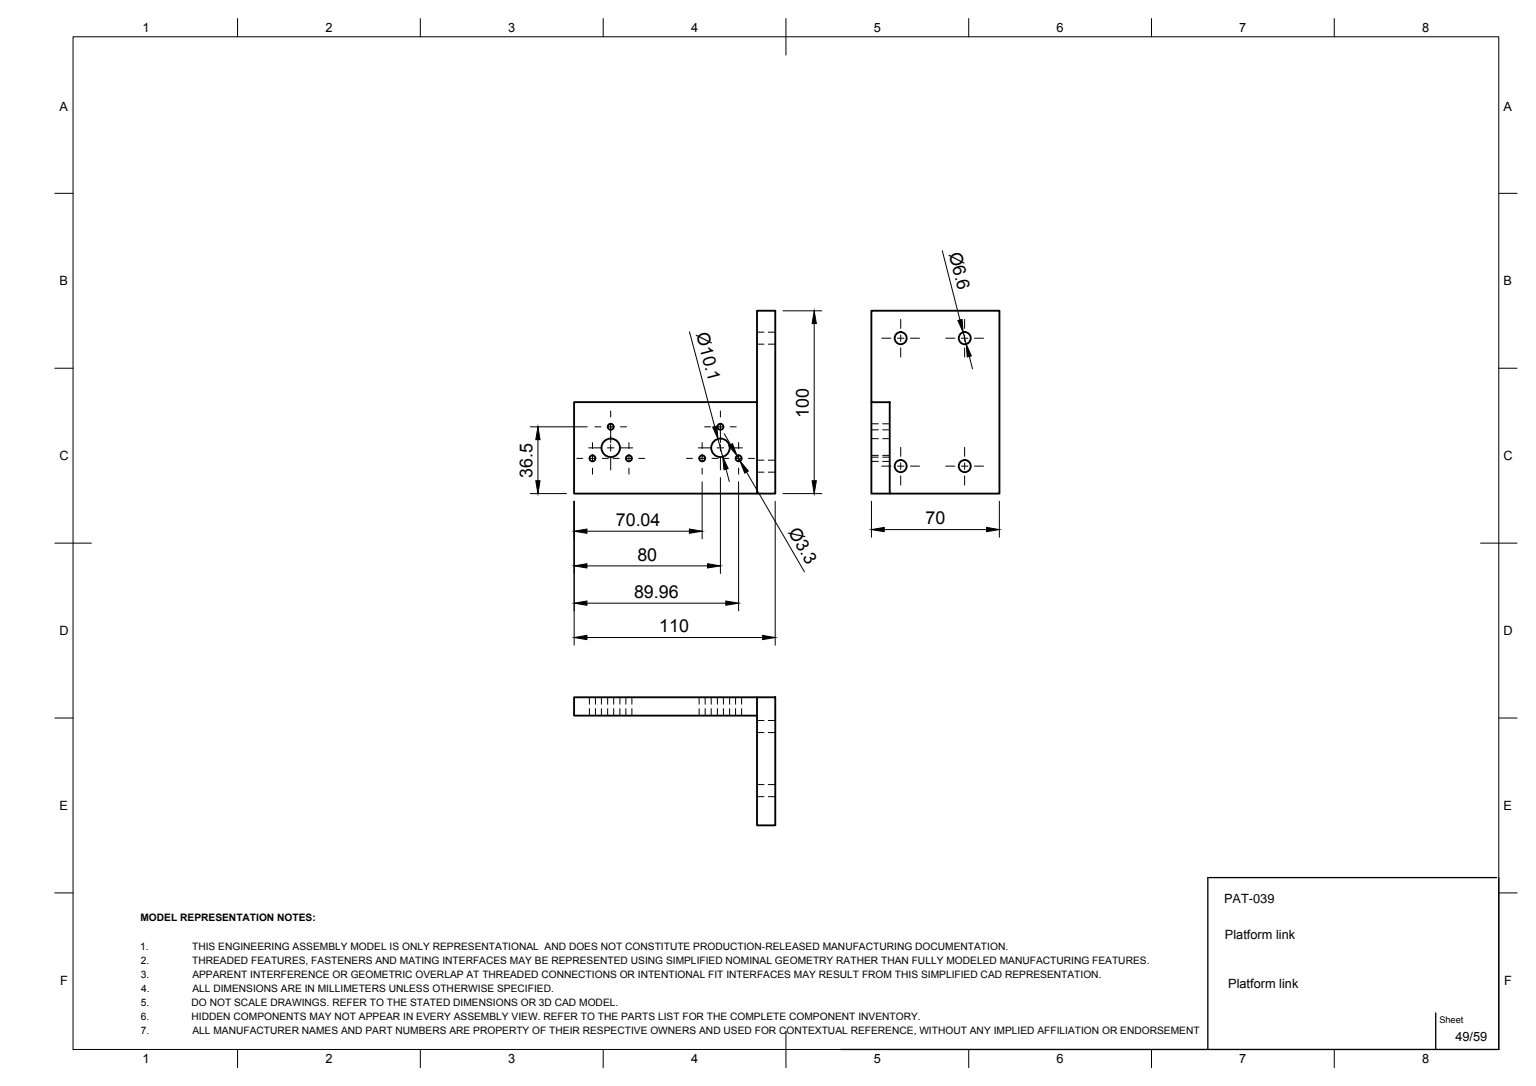
ISO-10303-21;
HEADER;
/* Generated by software containing ST-Developer
 * from STEP Tools, Inc. (www.steptools.com) 
 */

FILE_DESCRIPTION(
/* description */ ('Four-bar parallelogram arm'),
/* implementation_level */ '2;1');

FILE_NAME(
/* name */ 'Platform link.step',
/* time_stamp */ '2026-10-28T03:24:55-07:00',
/* author */ (''),
/* organization */ (''),
/* preprocessor_version */ 'ST-DEVELOPER v20.2',
/* originating_system */ 'Autodesk Translation Framework v15.17.0.0',
/* authorisation */ '');

FILE_SCHEMA (('AUTOMOTIVE_DESIGN { 1 0 10303 214 3 1 1 }'));
ENDSEC;

DATA;
#10=MECHANICAL_DESIGN_GEOMETRIC_PRESENTATION_REPRESENTATION('',(#668),#14512);
#560=SHAPE_REPRESENTATION_RELATIONSHIP('SRR','None',#14785,#610);
#610=ADVANCED_BREP_SHAPE_REPRESENTATION('',(#724),#14500);
#668=STYLED_ITEM('',(#15080),#724);
#724=MANIFOLD_SOLID_BREP('Body1',#7374);
#947=FACE_BOUND('',#2174,.T.);
#948=FACE_BOUND('',#2175,.T.);
#949=FACE_BOUND('',#2176,.T.);
#950=FACE_BOUND('',#2177,.T.);
#951=FACE_BOUND('',#2179,.T.);
#952=FACE_BOUND('',#2180,.T.);
#953=FACE_BOUND('',#2181,.T.);
#954=FACE_BOUND('',#2182,.T.);
#955=FACE_BOUND('',#2184,.T.);
#956=FACE_BOUND('',#2185,.T.);
#957=FACE_BOUND('',#2186,.T.);
#958=FACE_BOUND('',#2187,.T.);
#959=FACE_BOUND('',#2188,.T.);
#960=FACE_BOUND('',#2189,.T.);
#961=FACE_BOUND('',#2190,.T.);
#962=FACE_BOUND('',#2191,.T.);
#963=FACE_BOUND('',#2194,.T.);
#964=FACE_BOUND('',#2195,.T.);
#965=FACE_BOUND('',#2196,.T.);
#966=FACE_BOUND('',#2197,.T.);
#967=FACE_BOUND('',#2198,.T.);
#968=FACE_BOUND('',#2199,.T.);
#969=FACE_BOUND('',#2200,.T.);
#970=FACE_BOUND('',#2201,.T.);
#1155=PLANE('',#8757);
#1156=PLANE('',#8758);
#1157=PLANE('',#8759);
#1158=PLANE('',#8760);
#1159=PLANE('',#8761);
#1160=PLANE('',#8762);
#1161=PLANE('',#8763);
#1162=PLANE('',#8764);
#1163=PLANE('',#8765);
#1527=FACE_OUTER_BOUND('',#2159,.T.);
#1528=FACE_OUTER_BOUND('',#2160,.T.);
#1529=FACE_OUTER_BOUND('',#2161,.T.);
#1530=FACE_OUTER_BOUND('',#2162,.T.);
#1531=FACE_OUTER_BOUND('',#2163,.T.);
#1532=FACE_OUTER_BOUND('',#2164,.T.);
#1533=FACE_OUTER_BOUND('',#2165,.T.);
#1534=FACE_OUTER_BOUND('',#2166,.T.);
#1535=FACE_OUTER_BOUND('',#2167,.T.);
#1536=FACE_OUTER_BOUND('',#2168,.T.);
#1537=FACE_OUTER_BOUND('',#2169,.T.);
#1538=FACE_OUTER_BOUND('',#2170,.T.);
#1539=FACE_OUTER_BOUND('',#2171,.T.);
#1540=FACE_OUTER_BOUND('',#2172,.T.);
#1541=FACE_OUTER_BOUND('',#2173,.T.);
#1542=FACE_OUTER_BOUND('',#2178,.T.);
#1543=FACE_OUTER_BOUND('',#2183,.T.);
#1544=FACE_OUTER_BOUND('',#2192,.T.);
#1545=FACE_OUTER_BOUND('',#2193,.T.);
#1546=FACE_OUTER_BOUND('',#2202,.T.);
#1547=FACE_OUTER_BOUND('',#2203,.T.);
#2159=EDGE_LOOP('',(#6356,#6357,#6358,#6359));
#2160=EDGE_LOOP('',(#6360,#6361,#6362,#6363));
#2161=EDGE_LOOP('',(#6364,#6365,#6366,#6367));
#2162=EDGE_LOOP('',(#6368,#6369,#6370,#6371));
#2163=EDGE_LOOP('',(#6372,#6373,#6374,#6375));
#2164=EDGE_LOOP('',(#6376,#6377,#6378,#6379));
#2165=EDGE_LOOP('',(#6380,#6381,#6382,#6383));
#2166=EDGE_LOOP('',(#6384,#6385,#6386,#6387));
#2167=EDGE_LOOP('',(#6388,#6389,#6390,#6391));
#2168=EDGE_LOOP('',(#6392,#6393,#6394,#6395));
#2169=EDGE_LOOP('',(#6396,#6397,#6398,#6399));
#2170=EDGE_LOOP('',(#6400,#6401,#6402,#6403));
#2171=EDGE_LOOP('',(#6404,#6405,#6406,#6407));
#2172=EDGE_LOOP('',(#6408,#6409,#6410,#6411));
#2173=EDGE_LOOP('',(#6412,#6413,#6414,#6415));
#2174=EDGE_LOOP('',(#6416));
#2175=EDGE_LOOP('',(#6417));
#2176=EDGE_LOOP('',(#6418));
#2177=EDGE_LOOP('',(#6419));
#2178=EDGE_LOOP('',(#6420,#6421,#6422,#6423,#6424,#6425));
#2179=EDGE_LOOP('',(#6426));
#2180=EDGE_LOOP('',(#6427));
#2181=EDGE_LOOP('',(#6428));
#2182=EDGE_LOOP('',(#6429));
#2183=EDGE_LOOP('',(#6430,#6431,#6432,#6433));
#2184=EDGE_LOOP('',(#6434));
#2185=EDGE_LOOP('',(#6435));
#2186=EDGE_LOOP('',(#6436));
#2187=EDGE_LOOP('',(#6437));
#2188=EDGE_LOOP('',(#6438));
#2189=EDGE_LOOP('',(#6439));
#2190=EDGE_LOOP('',(#6440));
#2191=EDGE_LOOP('',(#6441));
#2192=EDGE_LOOP('',(#6442,#6443,#6444,#6445));
#2193=EDGE_LOOP('',(#6446,#6447,#6448,#6449,#6450,#6451));
#2194=EDGE_LOOP('',(#6452));
#2195=EDGE_LOOP('',(#6453));
#2196=EDGE_LOOP('',(#6454));
#2197=EDGE_LOOP('',(#6455));
#2198=EDGE_LOOP('',(#6456));
#2199=EDGE_LOOP('',(#6457));
#2200=EDGE_LOOP('',(#6458));
#2201=EDGE_LOOP('',(#6459));
#2202=EDGE_LOOP('',(#6460,#6461,#6462,#6463,#6464,#6465));
#2203=EDGE_LOOP('',(#6466,#6467,#6468,#6469));
#2619=LINE('',#13949,#3013);
#2620=LINE('',#13955,#3014);
#2621=LINE('',#13961,#3015);
#2622=LINE('',#13967,#3016);
#2623=LINE('',#13973,#3017);
#2624=LINE('',#13979,#3018);
#2625=LINE('',#13985,#3019);
#2626=LINE('',#13991,#3020);
#2627=LINE('',#13997,#3021);
#2628=LINE('',#14003,#3022);
#2629=LINE('',#14009,#3023);
#2630=LINE('',#14015,#3024);
#2631=LINE('',#14020,#3025);
#2632=LINE('',#14022,#3026);
#2633=LINE('',#14024,#3027);
#2634=LINE('',#14025,#3028);
#2635=LINE('',#14028,#3029);
#2636=LINE('',#14030,#3030);
#2637=LINE('',#14031,#3031);
#2638=LINE('',#14034,#3032);
#2639=LINE('',#14035,#3033);
#2640=LINE('',#14039,#3034);
#2641=LINE('',#14040,#3035);
#2642=LINE('',#14042,#3036);
#2643=LINE('',#14043,#3037);
#2644=LINE('',#14047,#3038);
#2645=LINE('',#14048,#3039);
#2646=LINE('',#14049,#3040);
#2647=LINE('',#14052,#3041);
#2648=LINE('',#14053,#3042);
#2649=LINE('',#14056,#3043);
#2650=LINE('',#14057,#3044);
#2651=LINE('',#14059,#3045);
#3013=VECTOR('',#10847,0.164999999999999);
#3014=VECTOR('',#10854,0.164999999999999);
#3015=VECTOR('',#10861,0.164999999999999);
#3016=VECTOR('',#10868,0.504999999999999);
#3017=VECTOR('',#10875,0.164999999999999);
#3018=VECTOR('',#10882,0.164999999999999);
#3019=VECTOR('',#10889,0.164999999999999);
#3020=VECTOR('',#10896,0.504999999999999);
#3021=VECTOR('',#10903,0.329999999999998);
#3022=VECTOR('',#10910,0.329999999999998);
#3023=VECTOR('',#10917,0.329999999999998);
#3024=VECTOR('',#10924,0.329999999999998);
#3025=VECTOR('',#10929,1.);
#3026=VECTOR('',#10930,1.);
#3027=VECTOR('',#10931,1.);
#3028=VECTOR('',#10932,1.);
#3029=VECTOR('',#10935,1.);
#3030=VECTOR('',#10936,1.);
#3031=VECTOR('',#10937,1.);
#3032=VECTOR('',#10940,1.);
#3033=VECTOR('',#10941,1.);
#3034=VECTOR('',#10944,1.);
#3035=VECTOR('',#10945,1.);
#3036=VECTOR('',#10946,1.);
#3037=VECTOR('',#10947,1.);
#3038=VECTOR('',#10950,1.);
#3039=VECTOR('',#10951,1.);
#3040=VECTOR('',#10952,1.);
#3041=VECTOR('',#10955,1.);
#3042=VECTOR('',#10956,1.);
#3043=VECTOR('',#10959,1.);
#3044=VECTOR('',#10960,1.);
#3045=VECTOR('',#10963,1.);
#3453=CIRCLE('',#8722,0.164999999999999);
#3454=CIRCLE('',#8723,0.164999999999999);
#3455=CIRCLE('',#8725,0.164999999999999);
#3456=CIRCLE('',#8726,0.164999999999999);
#3457=CIRCLE('',#8728,0.164999999999999);
#3458=CIRCLE('',#8729,0.164999999999999);
#3459=CIRCLE('',#8731,0.504999999999999);
#3460=CIRCLE('',#8732,0.504999999999999);
#3461=CIRCLE('',#8734,0.164999999999999);
#3462=CIRCLE('',#8735,0.164999999999999);
#3463=CIRCLE('',#8737,0.164999999999999);
#3464=CIRCLE('',#8738,0.164999999999999);
#3465=CIRCLE('',#8740,0.164999999999999);
#3466=CIRCLE('',#8741,0.164999999999999);
#3467=CIRCLE('',#8743,0.504999999999999);
#3468=CIRCLE('',#8744,0.504999999999999);
#3469=CIRCLE('',#8746,0.329999999999998);
#3470=CIRCLE('',#8747,0.329999999999998);
#3471=CIRCLE('',#8749,0.329999999999998);
#3472=CIRCLE('',#8750,0.329999999999998);
#3473=CIRCLE('',#8752,0.329999999999998);
#3474=CIRCLE('',#8753,0.329999999999998);
#3475=CIRCLE('',#8755,0.329999999999998);
#3476=CIRCLE('',#8756,0.329999999999998);
#4007=VERTEX_POINT('',#13946);
#4008=VERTEX_POINT('',#13948);
#4009=VERTEX_POINT('',#13952);
#4010=VERTEX_POINT('',#13954);
#4011=VERTEX_POINT('',#13958);
#4012=VERTEX_POINT('',#13960);
#4013=VERTEX_POINT('',#13964);
#4014=VERTEX_POINT('',#13966);
#4015=VERTEX_POINT('',#13970);
#4016=VERTEX_POINT('',#13972);
#4017=VERTEX_POINT('',#13976);
#4018=VERTEX_POINT('',#13978);
#4019=VERTEX_POINT('',#13982);
#4020=VERTEX_POINT('',#13984);
#4021=VERTEX_POINT('',#13988);
#4022=VERTEX_POINT('',#13990);
#4023=VERTEX_POINT('',#13994);
#4024=VERTEX_POINT('',#13996);
#4025=VERTEX_POINT('',#14000);
#4026=VERTEX_POINT('',#14002);
#4027=VERTEX_POINT('',#14006);
#4028=VERTEX_POINT('',#14008);
#4029=VERTEX_POINT('',#14012);
#4030=VERTEX_POINT('',#14014);
#4031=VERTEX_POINT('',#14018);
#4032=VERTEX_POINT('',#14019);
#4033=VERTEX_POINT('',#14021);
#4034=VERTEX_POINT('',#14023);
#4035=VERTEX_POINT('',#14027);
#4036=VERTEX_POINT('',#14029);
#4037=VERTEX_POINT('',#14033);
#4038=VERTEX_POINT('',#14037);
#4039=VERTEX_POINT('',#14038);
#4040=VERTEX_POINT('',#14041);
#4041=VERTEX_POINT('',#14045);
#4042=VERTEX_POINT('',#14046);
#4043=VERTEX_POINT('',#14051);
#4044=VERTEX_POINT('',#14055);
#4809=EDGE_CURVE('',#4007,#4007,#3453,.T.);
#4810=EDGE_CURVE('',#4007,#4008,#2619,.T.);
#4811=EDGE_CURVE('',#4008,#4008,#3454,.T.);
#4812=EDGE_CURVE('',#4009,#4009,#3455,.T.);
#4813=EDGE_CURVE('',#4009,#4010,#2620,.T.);
#4814=EDGE_CURVE('',#4010,#4010,#3456,.T.);
#4815=EDGE_CURVE('',#4011,#4011,#3457,.T.);
#4816=EDGE_CURVE('',#4011,#4012,#2621,.T.);
#4817=EDGE_CURVE('',#4012,#4012,#3458,.T.);
#4818=EDGE_CURVE('',#4013,#4013,#3459,.T.);
#4819=EDGE_CURVE('',#4013,#4014,#2622,.T.);
#4820=EDGE_CURVE('',#4014,#4014,#3460,.T.);
#4821=EDGE_CURVE('',#4015,#4015,#3461,.T.);
#4822=EDGE_CURVE('',#4015,#4016,#2623,.T.);
#4823=EDGE_CURVE('',#4016,#4016,#3462,.T.);
#4824=EDGE_CURVE('',#4017,#4017,#3463,.T.);
#4825=EDGE_CURVE('',#4017,#4018,#2624,.T.);
#4826=EDGE_CURVE('',#4018,#4018,#3464,.T.);
#4827=EDGE_CURVE('',#4019,#4019,#3465,.T.);
#4828=EDGE_CURVE('',#4019,#4020,#2625,.T.);
#4829=EDGE_CURVE('',#4020,#4020,#3466,.T.);
#4830=EDGE_CURVE('',#4021,#4021,#3467,.T.);
#4831=EDGE_CURVE('',#4021,#4022,#2626,.T.);
#4832=EDGE_CURVE('',#4022,#4022,#3468,.T.);
#4833=EDGE_CURVE('',#4023,#4023,#3469,.T.);
#4834=EDGE_CURVE('',#4023,#4024,#2627,.T.);
#4835=EDGE_CURVE('',#4024,#4024,#3470,.T.);
#4836=EDGE_CURVE('',#4025,#4025,#3471,.T.);
#4837=EDGE_CURVE('',#4025,#4026,#2628,.T.);
#4838=EDGE_CURVE('',#4026,#4026,#3472,.T.);
#4839=EDGE_CURVE('',#4027,#4027,#3473,.T.);
#4840=EDGE_CURVE('',#4027,#4028,#2629,.T.);
#4841=EDGE_CURVE('',#4028,#4028,#3474,.T.);
#4842=EDGE_CURVE('',#4029,#4029,#3475,.T.);
#4843=EDGE_CURVE('',#4029,#4030,#2630,.T.);
#4844=EDGE_CURVE('',#4030,#4030,#3476,.T.);
#4845=EDGE_CURVE('',#4031,#4032,#2631,.T.);
#4846=EDGE_CURVE('',#4032,#4033,#2632,.T.);
#4847=EDGE_CURVE('',#4034,#4033,#2633,.T.);
#4848=EDGE_CURVE('',#4031,#4034,#2634,.T.);
#4849=EDGE_CURVE('',#4035,#4031,#2635,.T.);
#4850=EDGE_CURVE('',#4036,#4034,#2636,.T.);
#4851=EDGE_CURVE('',#4035,#4036,#2637,.T.);
#4852=EDGE_CURVE('',#4033,#4037,#2638,.T.);
#4853=EDGE_CURVE('',#4037,#4036,#2639,.T.);
#4854=EDGE_CURVE('',#4038,#4039,#2640,.T.);
#4855=EDGE_CURVE('',#4032,#4039,#2641,.T.);
#4856=EDGE_CURVE('',#4040,#4035,#2642,.T.);
#4857=EDGE_CURVE('',#4040,#4038,#2643,.T.);
#4858=EDGE_CURVE('',#4041,#4042,#2644,.T.);
#4859=EDGE_CURVE('',#4042,#4039,#2645,.T.);
#4860=EDGE_CURVE('',#4041,#4038,#2646,.T.);
#4861=EDGE_CURVE('',#4043,#4041,#2647,.T.);
#4862=EDGE_CURVE('',#4043,#4040,#2648,.T.);
#4863=EDGE_CURVE('',#4044,#4043,#2649,.T.);
#4864=EDGE_CURVE('',#4044,#4037,#2650,.T.);
#4865=EDGE_CURVE('',#4042,#4044,#2651,.T.);
#6356=ORIENTED_EDGE('',*,*,#4809,.F.);
#6357=ORIENTED_EDGE('',*,*,#4810,.T.);
#6358=ORIENTED_EDGE('',*,*,#4811,.F.);
#6359=ORIENTED_EDGE('',*,*,#4810,.F.);
#6360=ORIENTED_EDGE('',*,*,#4812,.F.);
#6361=ORIENTED_EDGE('',*,*,#4813,.T.);
#6362=ORIENTED_EDGE('',*,*,#4814,.F.);
#6363=ORIENTED_EDGE('',*,*,#4813,.F.);
#6364=ORIENTED_EDGE('',*,*,#4815,.F.);
#6365=ORIENTED_EDGE('',*,*,#4816,.T.);
#6366=ORIENTED_EDGE('',*,*,#4817,.F.);
#6367=ORIENTED_EDGE('',*,*,#4816,.F.);
#6368=ORIENTED_EDGE('',*,*,#4818,.F.);
#6369=ORIENTED_EDGE('',*,*,#4819,.T.);
#6370=ORIENTED_EDGE('',*,*,#4820,.F.);
#6371=ORIENTED_EDGE('',*,*,#4819,.F.);
#6372=ORIENTED_EDGE('',*,*,#4821,.F.);
#6373=ORIENTED_EDGE('',*,*,#4822,.T.);
#6374=ORIENTED_EDGE('',*,*,#4823,.F.);
#6375=ORIENTED_EDGE('',*,*,#4822,.F.);
#6376=ORIENTED_EDGE('',*,*,#4824,.F.);
#6377=ORIENTED_EDGE('',*,*,#4825,.T.);
#6378=ORIENTED_EDGE('',*,*,#4826,.F.);
#6379=ORIENTED_EDGE('',*,*,#4825,.F.);
#6380=ORIENTED_EDGE('',*,*,#4827,.F.);
#6381=ORIENTED_EDGE('',*,*,#4828,.T.);
#6382=ORIENTED_EDGE('',*,*,#4829,.F.);
#6383=ORIENTED_EDGE('',*,*,#4828,.F.);
#6384=ORIENTED_EDGE('',*,*,#4830,.F.);
#6385=ORIENTED_EDGE('',*,*,#4831,.T.);
#6386=ORIENTED_EDGE('',*,*,#4832,.F.);
#6387=ORIENTED_EDGE('',*,*,#4831,.F.);
#6388=ORIENTED_EDGE('',*,*,#4833,.F.);
#6389=ORIENTED_EDGE('',*,*,#4834,.T.);
#6390=ORIENTED_EDGE('',*,*,#4835,.F.);
#6391=ORIENTED_EDGE('',*,*,#4834,.F.);
#6392=ORIENTED_EDGE('',*,*,#4836,.F.);
#6393=ORIENTED_EDGE('',*,*,#4837,.T.);
#6394=ORIENTED_EDGE('',*,*,#4838,.F.);
#6395=ORIENTED_EDGE('',*,*,#4837,.F.);
#6396=ORIENTED_EDGE('',*,*,#4839,.F.);
#6397=ORIENTED_EDGE('',*,*,#4840,.T.);
#6398=ORIENTED_EDGE('',*,*,#4841,.F.);
#6399=ORIENTED_EDGE('',*,*,#4840,.F.);
#6400=ORIENTED_EDGE('',*,*,#4842,.F.);
#6401=ORIENTED_EDGE('',*,*,#4843,.T.);
#6402=ORIENTED_EDGE('',*,*,#4844,.F.);
#6403=ORIENTED_EDGE('',*,*,#4843,.F.);
#6404=ORIENTED_EDGE('',*,*,#4845,.T.);
#6405=ORIENTED_EDGE('',*,*,#4846,.T.);
#6406=ORIENTED_EDGE('',*,*,#4847,.F.);
#6407=ORIENTED_EDGE('',*,*,#4848,.F.);
#6408=ORIENTED_EDGE('',*,*,#4849,.T.);
#6409=ORIENTED_EDGE('',*,*,#4848,.T.);
#6410=ORIENTED_EDGE('',*,*,#4850,.F.);
#6411=ORIENTED_EDGE('',*,*,#4851,.F.);
#6412=ORIENTED_EDGE('',*,*,#4852,.T.);
#6413=ORIENTED_EDGE('',*,*,#4853,.T.);
#6414=ORIENTED_EDGE('',*,*,#4850,.T.);
#6415=ORIENTED_EDGE('',*,*,#4847,.T.);
#6416=ORIENTED_EDGE('',*,*,#4835,.T.);
#6417=ORIENTED_EDGE('',*,*,#4838,.T.);
#6418=ORIENTED_EDGE('',*,*,#4841,.T.);
#6419=ORIENTED_EDGE('',*,*,#4844,.T.);
#6420=ORIENTED_EDGE('',*,*,#4854,.T.);
#6421=ORIENTED_EDGE('',*,*,#4855,.F.);
#6422=ORIENTED_EDGE('',*,*,#4845,.F.);
#6423=ORIENTED_EDGE('',*,*,#4849,.F.);
#6424=ORIENTED_EDGE('',*,*,#4856,.F.);
#6425=ORIENTED_EDGE('',*,*,#4857,.T.);
#6426=ORIENTED_EDGE('',*,*,#4833,.T.);
#6427=ORIENTED_EDGE('',*,*,#4836,.T.);
#6428=ORIENTED_EDGE('',*,*,#4839,.T.);
#6429=ORIENTED_EDGE('',*,*,#4842,.T.);
#6430=ORIENTED_EDGE('',*,*,#4858,.T.);
#6431=ORIENTED_EDGE('',*,*,#4859,.T.);
#6432=ORIENTED_EDGE('',*,*,#4854,.F.);
#6433=ORIENTED_EDGE('',*,*,#4860,.F.);
#6434=ORIENTED_EDGE('',*,*,#4832,.T.);
#6435=ORIENTED_EDGE('',*,*,#4829,.T.);
#6436=ORIENTED_EDGE('',*,*,#4826,.T.);
#6437=ORIENTED_EDGE('',*,*,#4823,.T.);
#6438=ORIENTED_EDGE('',*,*,#4820,.T.);
#6439=ORIENTED_EDGE('',*,*,#4817,.T.);
#6440=ORIENTED_EDGE('',*,*,#4814,.T.);
#6441=ORIENTED_EDGE('',*,*,#4811,.T.);
#6442=ORIENTED_EDGE('',*,*,#4861,.T.);
#6443=ORIENTED_EDGE('',*,*,#4860,.T.);
#6444=ORIENTED_EDGE('',*,*,#4857,.F.);
#6445=ORIENTED_EDGE('',*,*,#4862,.F.);
#6446=ORIENTED_EDGE('',*,*,#4863,.T.);
#6447=ORIENTED_EDGE('',*,*,#4862,.T.);
#6448=ORIENTED_EDGE('',*,*,#4856,.T.);
#6449=ORIENTED_EDGE('',*,*,#4851,.T.);
#6450=ORIENTED_EDGE('',*,*,#4853,.F.);
#6451=ORIENTED_EDGE('',*,*,#4864,.F.);
#6452=ORIENTED_EDGE('',*,*,#4830,.T.);
#6453=ORIENTED_EDGE('',*,*,#4827,.T.);
#6454=ORIENTED_EDGE('',*,*,#4824,.T.);
#6455=ORIENTED_EDGE('',*,*,#4821,.T.);
#6456=ORIENTED_EDGE('',*,*,#4818,.T.);
#6457=ORIENTED_EDGE('',*,*,#4815,.T.);
#6458=ORIENTED_EDGE('',*,*,#4812,.T.);
#6459=ORIENTED_EDGE('',*,*,#4809,.T.);
#6460=ORIENTED_EDGE('',*,*,#4865,.T.);
#6461=ORIENTED_EDGE('',*,*,#4864,.T.);
#6462=ORIENTED_EDGE('',*,*,#4852,.F.);
#6463=ORIENTED_EDGE('',*,*,#4846,.F.);
#6464=ORIENTED_EDGE('',*,*,#4855,.T.);
#6465=ORIENTED_EDGE('',*,*,#4859,.F.);
#6466=ORIENTED_EDGE('',*,*,#4865,.F.);
#6467=ORIENTED_EDGE('',*,*,#4858,.F.);
#6468=ORIENTED_EDGE('',*,*,#4861,.F.);
#6469=ORIENTED_EDGE('',*,*,#4863,.F.);
#6862=CYLINDRICAL_SURFACE('',#8721,0.164999999999999);
#6863=CYLINDRICAL_SURFACE('',#8724,0.164999999999999);
#6864=CYLINDRICAL_SURFACE('',#8727,0.164999999999999);
#6865=CYLINDRICAL_SURFACE('',#8730,0.504999999999999);
#6866=CYLINDRICAL_SURFACE('',#8733,0.164999999999999);
#6867=CYLINDRICAL_SURFACE('',#8736,0.164999999999999);
#6868=CYLINDRICAL_SURFACE('',#8739,0.164999999999999);
#6869=CYLINDRICAL_SURFACE('',#8742,0.504999999999999);
#6870=CYLINDRICAL_SURFACE('',#8745,0.329999999999998);
#6871=CYLINDRICAL_SURFACE('',#8748,0.329999999999998);
#6872=CYLINDRICAL_SURFACE('',#8751,0.329999999999998);
#6873=CYLINDRICAL_SURFACE('',#8754,0.329999999999998);
#7232=ADVANCED_FACE('',(#1527),#6862,.F.);
#7233=ADVANCED_FACE('',(#1528),#6863,.F.);
#7234=ADVANCED_FACE('',(#1529),#6864,.F.);
#7235=ADVANCED_FACE('',(#1530),#6865,.F.);
#7236=ADVANCED_FACE('',(#1531),#6866,.F.);
#7237=ADVANCED_FACE('',(#1532),#6867,.F.);
#7238=ADVANCED_FACE('',(#1533),#6868,.F.);
#7239=ADVANCED_FACE('',(#1534),#6869,.F.);
#7240=ADVANCED_FACE('',(#1535),#6870,.F.);
#7241=ADVANCED_FACE('',(#1536),#6871,.F.);
#7242=ADVANCED_FACE('',(#1537),#6872,.F.);
#7243=ADVANCED_FACE('',(#1538),#6873,.F.);
#7244=ADVANCED_FACE('',(#1539),#1155,.T.);
#7245=ADVANCED_FACE('',(#1540),#1156,.T.);
#7246=ADVANCED_FACE('',(#1541,#947,#948,#949,#950),#1157,.T.);
#7247=ADVANCED_FACE('',(#1542,#951,#952,#953,#954),#1158,.F.);
#7248=ADVANCED_FACE('',(#1543,#955,#956,#957,#958,#959,#960,#961,#962),
#1159,.T.);
#7249=ADVANCED_FACE('',(#1544),#1160,.T.);
#7250=ADVANCED_FACE('',(#1545,#963,#964,#965,#966,#967,#968,#969,#970),
#1161,.T.);
#7251=ADVANCED_FACE('',(#1546),#1162,.T.);
#7252=ADVANCED_FACE('',(#1547),#1163,.F.);
#7374=CLOSED_SHELL('',(#7232,#7233,#7234,#7235,#7236,#7237,#7238,#7239,
#7240,#7241,#7242,#7243,#7244,#7245,#7246,#7247,#7248,#7249,#7250,#7251,
#7252));
#8720=AXIS2_PLACEMENT_3D('',#13944,#10841,#10842);
#8721=AXIS2_PLACEMENT_3D('',#13945,#10843,#10844);
#8722=AXIS2_PLACEMENT_3D('',#13947,#10845,#10846);
#8723=AXIS2_PLACEMENT_3D('',#13950,#10848,#10849);
#8724=AXIS2_PLACEMENT_3D('',#13951,#10850,#10851);
#8725=AXIS2_PLACEMENT_3D('',#13953,#10852,#10853);
#8726=AXIS2_PLACEMENT_3D('',#13956,#10855,#10856);
#8727=AXIS2_PLACEMENT_3D('',#13957,#10857,#10858);
#8728=AXIS2_PLACEMENT_3D('',#13959,#10859,#10860);
#8729=AXIS2_PLACEMENT_3D('',#13962,#10862,#10863);
#8730=AXIS2_PLACEMENT_3D('',#13963,#10864,#10865);
#8731=AXIS2_PLACEMENT_3D('',#13965,#10866,#10867);
#8732=AXIS2_PLACEMENT_3D('',#13968,#10869,#10870);
#8733=AXIS2_PLACEMENT_3D('',#13969,#10871,#10872);
#8734=AXIS2_PLACEMENT_3D('',#13971,#10873,#10874);
#8735=AXIS2_PLACEMENT_3D('',#13974,#10876,#10877);
#8736=AXIS2_PLACEMENT_3D('',#13975,#10878,#10879);
#8737=AXIS2_PLACEMENT_3D('',#13977,#10880,#10881);
#8738=AXIS2_PLACEMENT_3D('',#13980,#10883,#10884);
#8739=AXIS2_PLACEMENT_3D('',#13981,#10885,#10886);
#8740=AXIS2_PLACEMENT_3D('',#13983,#10887,#10888);
#8741=AXIS2_PLACEMENT_3D('',#13986,#10890,#10891);
#8742=AXIS2_PLACEMENT_3D('',#13987,#10892,#10893);
#8743=AXIS2_PLACEMENT_3D('',#13989,#10894,#10895);
#8744=AXIS2_PLACEMENT_3D('',#13992,#10897,#10898);
#8745=AXIS2_PLACEMENT_3D('',#13993,#10899,#10900);
#8746=AXIS2_PLACEMENT_3D('',#13995,#10901,#10902);
#8747=AXIS2_PLACEMENT_3D('',#13998,#10904,#10905);
#8748=AXIS2_PLACEMENT_3D('',#13999,#10906,#10907);
#8749=AXIS2_PLACEMENT_3D('',#14001,#10908,#10909);
#8750=AXIS2_PLACEMENT_3D('',#14004,#10911,#10912);
#8751=AXIS2_PLACEMENT_3D('',#14005,#10913,#10914);
#8752=AXIS2_PLACEMENT_3D('',#14007,#10915,#10916);
#8753=AXIS2_PLACEMENT_3D('',#14010,#10918,#10919);
#8754=AXIS2_PLACEMENT_3D('',#14011,#10920,#10921);
#8755=AXIS2_PLACEMENT_3D('',#14013,#10922,#10923);
#8756=AXIS2_PLACEMENT_3D('',#14016,#10925,#10926);
#8757=AXIS2_PLACEMENT_3D('',#14017,#10927,#10928);
#8758=AXIS2_PLACEMENT_3D('',#14026,#10933,#10934);
#8759=AXIS2_PLACEMENT_3D('',#14032,#10938,#10939);
#8760=AXIS2_PLACEMENT_3D('',#14036,#10942,#10943);
#8761=AXIS2_PLACEMENT_3D('',#14044,#10948,#10949);
#8762=AXIS2_PLACEMENT_3D('',#14050,#10953,#10954);
#8763=AXIS2_PLACEMENT_3D('',#14054,#10957,#10958);
#8764=AXIS2_PLACEMENT_3D('',#14058,#10961,#10962);
#8765=AXIS2_PLACEMENT_3D('',#14060,#10964,#10965);
#10841=DIRECTION('axis',(0.,0.,1.));
#10842=DIRECTION('refdir',(1.,0.,0.));
#10843=DIRECTION('center_axis',(0.,1.,0.));
#10844=DIRECTION('ref_axis',(1.,0.,0.));
#10845=DIRECTION('center_axis',(0.,1.,0.));
#10846=DIRECTION('ref_axis',(1.,0.,0.));
#10847=DIRECTION('',(0.,1.,0.));
#10848=DIRECTION('center_axis',(0.,-1.,0.));
#10849=DIRECTION('ref_axis',(1.,0.,0.));
#10850=DIRECTION('center_axis',(0.,1.,0.));
#10851=DIRECTION('ref_axis',(1.,0.,0.));
#10852=DIRECTION('center_axis',(0.,1.,0.));
#10853=DIRECTION('ref_axis',(1.,0.,0.));
#10854=DIRECTION('',(0.,1.,0.));
#10855=DIRECTION('center_axis',(0.,-1.,0.));
#10856=DIRECTION('ref_axis',(1.,0.,0.));
#10857=DIRECTION('center_axis',(0.,1.,0.));
#10858=DIRECTION('ref_axis',(1.,0.,0.));
#10859=DIRECTION('center_axis',(0.,1.,0.));
#10860=DIRECTION('ref_axis',(1.,0.,0.));
#10861=DIRECTION('',(0.,1.,0.));
#10862=DIRECTION('center_axis',(0.,-1.,0.));
#10863=DIRECTION('ref_axis',(1.,0.,0.));
#10864=DIRECTION('center_axis',(0.,1.,0.));
#10865=DIRECTION('ref_axis',(1.,0.,0.));
#10866=DIRECTION('center_axis',(0.,1.,0.));
#10867=DIRECTION('ref_axis',(1.,0.,0.));
#10868=DIRECTION('',(0.,1.,0.));
#10869=DIRECTION('center_axis',(0.,-1.,0.));
#10870=DIRECTION('ref_axis',(1.,0.,0.));
#10871=DIRECTION('center_axis',(0.,1.,0.));
#10872=DIRECTION('ref_axis',(1.,0.,0.));
#10873=DIRECTION('center_axis',(0.,1.,0.));
#10874=DIRECTION('ref_axis',(1.,0.,0.));
#10875=DIRECTION('',(0.,1.,0.));
#10876=DIRECTION('center_axis',(0.,-1.,0.));
#10877=DIRECTION('ref_axis',(1.,0.,0.));
#10878=DIRECTION('center_axis',(0.,1.,0.));
#10879=DIRECTION('ref_axis',(1.,0.,0.));
#10880=DIRECTION('center_axis',(0.,1.,0.));
#10881=DIRECTION('ref_axis',(1.,0.,0.));
#10882=DIRECTION('',(0.,1.,0.));
#10883=DIRECTION('center_axis',(0.,-1.,0.));
#10884=DIRECTION('ref_axis',(1.,0.,0.));
#10885=DIRECTION('center_axis',(0.,1.,0.));
#10886=DIRECTION('ref_axis',(1.,0.,0.));
#10887=DIRECTION('center_axis',(0.,1.,0.));
#10888=DIRECTION('ref_axis',(1.,0.,0.));
#10889=DIRECTION('',(0.,1.,0.));
#10890=DIRECTION('center_axis',(0.,-1.,0.));
#10891=DIRECTION('ref_axis',(1.,0.,0.));
#10892=DIRECTION('center_axis',(0.,1.,0.));
#10893=DIRECTION('ref_axis',(1.,0.,0.));
#10894=DIRECTION('center_axis',(0.,1.,0.));
#10895=DIRECTION('ref_axis',(1.,0.,0.));
#10896=DIRECTION('',(0.,1.,0.));
#10897=DIRECTION('center_axis',(0.,-1.,0.));
#10898=DIRECTION('ref_axis',(1.,0.,0.));
#10899=DIRECTION('center_axis',(0.,0.,1.));
#10900=DIRECTION('ref_axis',(1.,0.,0.));
#10901=DIRECTION('center_axis',(0.,0.,1.));
#10902=DIRECTION('ref_axis',(1.,0.,0.));
#10903=DIRECTION('',(0.,0.,1.));
#10904=DIRECTION('center_axis',(0.,0.,-1.));
#10905=DIRECTION('ref_axis',(1.,0.,0.));
#10906=DIRECTION('center_axis',(0.,0.,1.));
#10907=DIRECTION('ref_axis',(1.,0.,0.));
#10908=DIRECTION('center_axis',(0.,0.,1.));
#10909=DIRECTION('ref_axis',(1.,0.,0.));
#10910=DIRECTION('',(0.,0.,1.));
#10911=DIRECTION('center_axis',(0.,0.,-1.));
#10912=DIRECTION('ref_axis',(1.,0.,0.));
#10913=DIRECTION('center_axis',(0.,0.,1.));
#10914=DIRECTION('ref_axis',(1.,0.,0.));
#10915=DIRECTION('center_axis',(0.,0.,1.));
#10916=DIRECTION('ref_axis',(1.,0.,0.));
#10917=DIRECTION('',(0.,0.,1.));
#10918=DIRECTION('center_axis',(0.,0.,-1.));
#10919=DIRECTION('ref_axis',(1.,0.,0.));
#10920=DIRECTION('center_axis',(0.,0.,1.));
#10921=DIRECTION('ref_axis',(1.,0.,0.));
#10922=DIRECTION('center_axis',(0.,0.,1.));
#10923=DIRECTION('ref_axis',(1.,0.,0.));
#10924=DIRECTION('',(0.,0.,1.));
#10925=DIRECTION('center_axis',(0.,0.,-1.));
#10926=DIRECTION('ref_axis',(1.,0.,0.));
#10927=DIRECTION('center_axis',(0.,1.,0.));
#10928=DIRECTION('ref_axis',(-1.,0.,0.));
#10929=DIRECTION('',(-1.,0.,0.));
#10930=DIRECTION('',(0.,0.,1.));
#10931=DIRECTION('',(-1.,0.,0.));
#10932=DIRECTION('',(0.,0.,1.));
#10933=DIRECTION('center_axis',(1.,0.,0.));
#10934=DIRECTION('ref_axis',(0.,1.,0.));
#10935=DIRECTION('',(0.,1.,0.));
#10936=DIRECTION('',(0.,1.,0.));
#10937=DIRECTION('',(0.,0.,1.));
#10938=DIRECTION('center_axis',(0.,0.,1.));
#10939=DIRECTION('ref_axis',(1.,0.,0.));
#10940=DIRECTION('',(0.,-1.,0.));
#10941=DIRECTION('',(1.,0.,0.));
#10942=DIRECTION('center_axis',(0.,0.,1.));
#10943=DIRECTION('ref_axis',(1.,0.,0.));
#10944=DIRECTION('',(-1.,0.,0.));
#10945=DIRECTION('',(0.,-1.,0.));
#10946=DIRECTION('',(1.,0.,0.));
#10947=DIRECTION('',(0.,1.,0.));
#10948=DIRECTION('center_axis',(0.,1.,0.));
#10949=DIRECTION('ref_axis',(-1.,0.,0.));
#10950=DIRECTION('',(-1.,0.,0.));
#10951=DIRECTION('',(0.,0.,1.));
#10952=DIRECTION('',(0.,0.,1.));
#10953=DIRECTION('center_axis',(1.,0.,0.));
#10954=DIRECTION('ref_axis',(0.,1.,0.));
#10955=DIRECTION('',(0.,1.,0.));
#10956=DIRECTION('',(0.,0.,1.));
#10957=DIRECTION('center_axis',(0.,-1.,0.));
#10958=DIRECTION('ref_axis',(1.,0.,0.));
#10959=DIRECTION('',(1.,0.,0.));
#10960=DIRECTION('',(0.,0.,1.));
#10961=DIRECTION('center_axis',(-1.,0.,0.));
#10962=DIRECTION('ref_axis',(0.,-1.,0.));
#10963=DIRECTION('',(0.,-1.,0.));
#10964=DIRECTION('center_axis',(0.,0.,1.));
#10965=DIRECTION('ref_axis',(1.,0.,0.));
#13944=CARTESIAN_POINT('',(0.,0.,0.));
#13945=CARTESIAN_POINT('Origin',(21.15,2.8,14.));
#13946=CARTESIAN_POINT('',(20.985,2.9,14.));
#13947=CARTESIAN_POINT('Origin',(21.15,2.9,14.));
#13948=CARTESIAN_POINT('',(20.985,3.9,14.));
#13949=CARTESIAN_POINT('',(20.985,2.8,14.));
#13950=CARTESIAN_POINT('Origin',(21.15,3.9,14.));
#13951=CARTESIAN_POINT('Origin',(19.425,2.8,14.9959292143521));
#13952=CARTESIAN_POINT('',(19.26,2.9,14.9959292143521));
#13953=CARTESIAN_POINT('Origin',(19.425,2.9,14.9959292143521));
#13954=CARTESIAN_POINT('',(19.26,3.9,14.9959292143521));
#13955=CARTESIAN_POINT('',(19.26,2.8,14.9959292143521));
#13956=CARTESIAN_POINT('Origin',(19.425,3.9,14.9959292143521));
#13957=CARTESIAN_POINT('Origin',(19.425,2.8,13.0040707856479));
#13958=CARTESIAN_POINT('',(19.26,2.9,13.0040707856479));
#13959=CARTESIAN_POINT('Origin',(19.425,2.9,13.0040707856479));
#13960=CARTESIAN_POINT('',(19.26,3.9,13.0040707856479));
#13961=CARTESIAN_POINT('',(19.26,2.8,13.0040707856479));
#13962=CARTESIAN_POINT('Origin',(19.425,3.9,13.0040707856479));
#13963=CARTESIAN_POINT('Origin',(20.,2.8,14.));
#13964=CARTESIAN_POINT('',(19.495,2.9,14.));
#13965=CARTESIAN_POINT('Origin',(20.,2.9,14.));
#13966=CARTESIAN_POINT('',(19.495,3.9,14.));
#13967=CARTESIAN_POINT('',(19.495,2.8,14.));
#13968=CARTESIAN_POINT('Origin',(20.,3.9,14.));
#13969=CARTESIAN_POINT('Origin',(21.15,2.8,8.));
#13970=CARTESIAN_POINT('',(20.985,2.9,8.));
#13971=CARTESIAN_POINT('Origin',(21.15,2.9,8.));
#13972=CARTESIAN_POINT('',(20.985,3.9,8.));
#13973=CARTESIAN_POINT('',(20.985,2.8,8.));
#13974=CARTESIAN_POINT('Origin',(21.15,3.9,8.));
#13975=CARTESIAN_POINT('Origin',(19.425,2.8,8.9959292143521));
#13976=CARTESIAN_POINT('',(19.26,2.9,8.9959292143521));
#13977=CARTESIAN_POINT('Origin',(19.425,2.9,8.9959292143521));
#13978=CARTESIAN_POINT('',(19.26,3.9,8.9959292143521));
#13979=CARTESIAN_POINT('',(19.26,2.8,8.9959292143521));
#13980=CARTESIAN_POINT('Origin',(19.425,3.9,8.9959292143521));
#13981=CARTESIAN_POINT('Origin',(19.425,2.8,7.0040707856479));
#13982=CARTESIAN_POINT('',(19.26,2.9,7.0040707856479));
#13983=CARTESIAN_POINT('Origin',(19.425,2.9,7.0040707856479));
#13984=CARTESIAN_POINT('',(19.26,3.9,7.0040707856479));
#13985=CARTESIAN_POINT('',(19.26,2.8,7.0040707856479));
#13986=CARTESIAN_POINT('Origin',(19.425,3.9,7.0040707856479));
#13987=CARTESIAN_POINT('Origin',(20.,2.8,8.));
#13988=CARTESIAN_POINT('',(19.495,2.9,8.));
#13989=CARTESIAN_POINT('Origin',(20.,2.9,8.));
#13990=CARTESIAN_POINT('',(19.495,3.9,8.));
#13991=CARTESIAN_POINT('',(19.495,2.8,8.));
#13992=CARTESIAN_POINT('Origin',(20.,3.9,8.));
#13993=CARTESIAN_POINT('Origin',(19.,8.,15.9));
#13994=CARTESIAN_POINT('',(18.67,8.,16.));
#13995=CARTESIAN_POINT('Origin',(19.,8.,16.));
#13996=CARTESIAN_POINT('',(18.67,8.,17.));
#13997=CARTESIAN_POINT('',(18.67,8.,15.9));
#13998=CARTESIAN_POINT('Origin',(19.,8.,17.));
#13999=CARTESIAN_POINT('Origin',(26.,4.5,15.9));
#14000=CARTESIAN_POINT('',(25.67,4.5,16.));
#14001=CARTESIAN_POINT('Origin',(26.,4.5,16.));
#14002=CARTESIAN_POINT('',(25.67,4.5,17.));
#14003=CARTESIAN_POINT('',(25.67,4.5,15.9));
#14004=CARTESIAN_POINT('Origin',(26.,4.5,17.));
#14005=CARTESIAN_POINT('Origin',(19.,4.5,15.9));
#14006=CARTESIAN_POINT('',(18.67,4.5,16.));
#14007=CARTESIAN_POINT('Origin',(19.,4.5,16.));
#14008=CARTESIAN_POINT('',(18.67,4.5,17.));
#14009=CARTESIAN_POINT('',(18.67,4.5,15.9));
#14010=CARTESIAN_POINT('Origin',(19.,4.5,17.));
#14011=CARTESIAN_POINT('Origin',(26.,8.,15.9));
#14012=CARTESIAN_POINT('',(25.67,8.,16.));
#14013=CARTESIAN_POINT('Origin',(26.,8.,16.));
#14014=CARTESIAN_POINT('',(25.67,8.,17.));
#14015=CARTESIAN_POINT('',(25.67,8.,15.9));
#14016=CARTESIAN_POINT('Origin',(26.,8.,17.));
#14017=CARTESIAN_POINT('Origin',(27.5,9.9,16.));
#14018=CARTESIAN_POINT('',(27.5,9.9,16.));
#14019=CARTESIAN_POINT('',(17.5,9.9,16.));
#14020=CARTESIAN_POINT('',(27.5,9.9,16.));
#14021=CARTESIAN_POINT('',(17.5,9.9,17.));
#14022=CARTESIAN_POINT('',(17.5,9.9,16.));
#14023=CARTESIAN_POINT('',(27.5,9.9,17.));
#14024=CARTESIAN_POINT('',(27.5,9.9,17.));
#14025=CARTESIAN_POINT('',(27.5,9.9,16.));
#14026=CARTESIAN_POINT('Origin',(27.5,2.9,16.));
#14027=CARTESIAN_POINT('',(27.5,2.9,16.));
#14028=CARTESIAN_POINT('',(27.5,2.9,16.));
#14029=CARTESIAN_POINT('',(27.5,2.9,17.));
#14030=CARTESIAN_POINT('',(27.5,2.9,17.));
#14031=CARTESIAN_POINT('',(27.5,2.9,16.));
#14032=CARTESIAN_POINT('Origin',(22.5,6.4,17.));
#14033=CARTESIAN_POINT('',(17.5,2.9,17.));
#14034=CARTESIAN_POINT('',(17.5,9.9,17.));
#14035=CARTESIAN_POINT('',(17.5,2.9,17.));
#14036=CARTESIAN_POINT('Origin',(22.5,6.4,16.));
#14037=CARTESIAN_POINT('',(22.5,3.9,16.));
#14038=CARTESIAN_POINT('',(17.5,3.9,16.));
#14039=CARTESIAN_POINT('',(22.5,3.9,16.));
#14040=CARTESIAN_POINT('',(17.5,9.9,16.));
#14041=CARTESIAN_POINT('',(22.5,2.9,16.));
#14042=CARTESIAN_POINT('',(17.5,2.9,16.));
#14043=CARTESIAN_POINT('',(22.5,2.9,16.));
#14044=CARTESIAN_POINT('Origin',(22.5,3.9,6.));
#14045=CARTESIAN_POINT('',(22.5,3.9,6.));
#14046=CARTESIAN_POINT('',(17.5,3.9,6.));
#14047=CARTESIAN_POINT('',(22.5,3.9,6.));
#14048=CARTESIAN_POINT('',(17.5,3.9,6.));
#14049=CARTESIAN_POINT('',(22.5,3.9,6.));
#14050=CARTESIAN_POINT('Origin',(22.5,2.9,6.));
#14051=CARTESIAN_POINT('',(22.5,2.9,6.));
#14052=CARTESIAN_POINT('',(22.5,2.9,6.));
#14053=CARTESIAN_POINT('',(22.5,2.9,6.));
#14054=CARTESIAN_POINT('Origin',(17.5,2.9,6.));
#14055=CARTESIAN_POINT('',(17.5,2.9,6.));
#14056=CARTESIAN_POINT('',(17.5,2.9,6.));
#14057=CARTESIAN_POINT('',(17.5,2.9,6.));
#14058=CARTESIAN_POINT('Origin',(17.5,3.9,6.));
#14059=CARTESIAN_POINT('',(17.5,3.9,6.));
#14060=CARTESIAN_POINT('Origin',(20.,3.4,6.));
#14443=UNCERTAINTY_MEASURE_WITH_UNIT(LENGTH_MEASURE(0.001),#14513,
'DISTANCE_ACCURACY_VALUE',
'Maximum model space distance between geometric entities at asserted c
onnectivities');
#14455=UNCERTAINTY_MEASURE_WITH_UNIT(LENGTH_MEASURE(0.001),#14513,
'DISTANCE_ACCURACY_VALUE',
'Maximum model space distance between geometric entities at asserted c
onnectivities');
#14500=(
GEOMETRIC_REPRESENTATION_CONTEXT(3)
GLOBAL_UNCERTAINTY_ASSIGNED_CONTEXT((#14443))
GLOBAL_UNIT_ASSIGNED_CONTEXT((#14513,#14515,#14516))
REPRESENTATION_CONTEXT('','3D')
);
#14512=(
GEOMETRIC_REPRESENTATION_CONTEXT(3)
GLOBAL_UNCERTAINTY_ASSIGNED_CONTEXT((#14455))
GLOBAL_UNIT_ASSIGNED_CONTEXT((#14513,#14515,#14516))
REPRESENTATION_CONTEXT('','3D')
);
#14513=(
LENGTH_UNIT()
NAMED_UNIT(*)
SI_UNIT(.CENTI.,.METRE.)
);
#14515=(
NAMED_UNIT(*)
PLANE_ANGLE_UNIT()
SI_UNIT($,.RADIAN.)
);
#14516=(
NAMED_UNIT(*)
SI_UNIT($,.STERADIAN.)
SOLID_ANGLE_UNIT()
);
#14561=SHAPE_DEFINITION_REPRESENTATION(#14677,#14785);
#14677=PRODUCT_DEFINITION_SHAPE('',$,#14842);
#14785=SHAPE_REPRESENTATION('',(#8720),#14500);
#14797=PRODUCT_DEFINITION_CONTEXT('part definition',#14967,'design');
#14842=PRODUCT_DEFINITION('Platform link','Platform link',#14898,#14797);
#14898=PRODUCT_DEFINITION_FORMATION('',$,#15013);
#14967=APPLICATION_CONTEXT(
'Core Data for Automotive Mechanical Design Process');
#14968=PRODUCT_CONTEXT('part definition',#14967,'mechanical');
#15013=PRODUCT('Platform link','Platform link','Platform link',(#14968));
#15074=COLOUR_RGB('Sky Blue',0.24,0.69,0.87);
#15075=FILL_AREA_STYLE_COLOUR('',#15074);
#15076=FILL_AREA_STYLE('',(#15075));
#15077=SURFACE_STYLE_FILL_AREA(#15076);
#15078=SURFACE_SIDE_STYLE('',(#15077));
#15079=SURFACE_STYLE_USAGE(.BOTH.,#15078);
#15080=PRESENTATION_STYLE_ASSIGNMENT((#15079));
ENDSEC;
END-ISO-10303-21;
